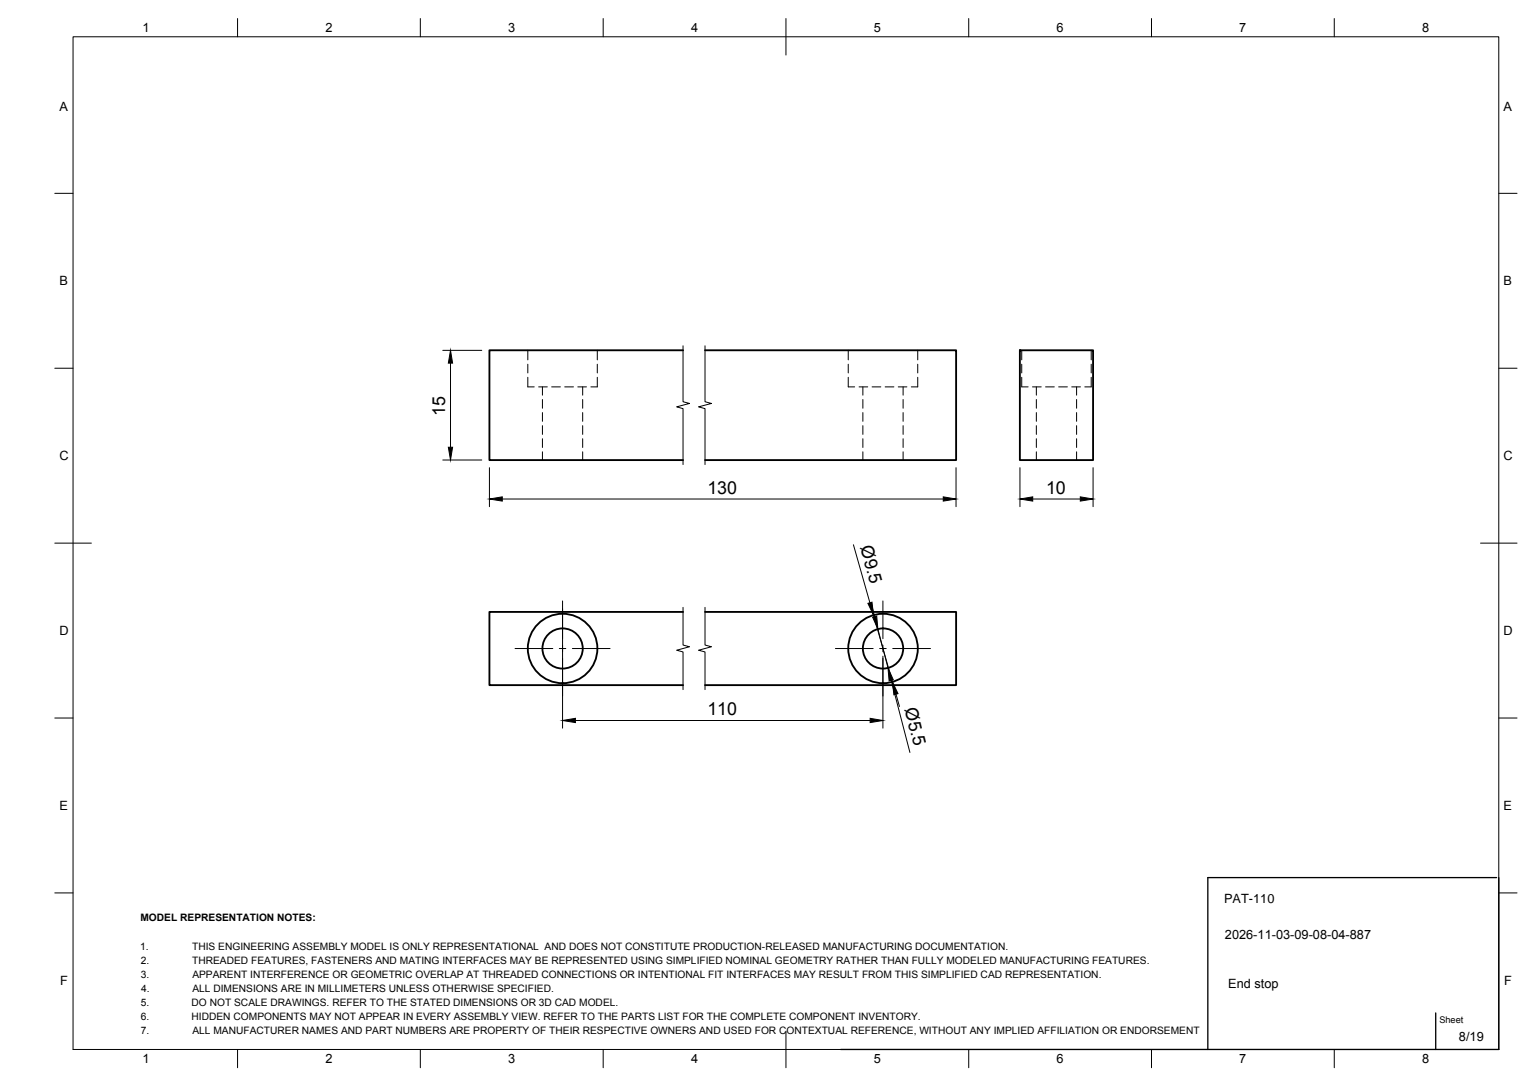
ISO-10303-21;
HEADER;
/* Generated by software containing ST-Developer
 * from STEP Tools, Inc. (www.steptools.com) 
 */

FILE_DESCRIPTION(
/* description */ ('Twin-shaft manual slide'),
/* implementation_level */ '2;1');

FILE_NAME(
/* name */ 'End stop.step',
/* time_stamp */ '2026-10-27T18:38:08-07:00',
/* author */ (''),
/* organization */ (''),
/* preprocessor_version */ 'ST-DEVELOPER v20.2',
/* originating_system */ 'Autodesk Translation Framework v15.17.0.0',
/* authorisation */ '');

FILE_SCHEMA (('AUTOMOTIVE_DESIGN { 1 0 10303 214 3 1 1 }'));
ENDSEC;

DATA;
#10=MECHANICAL_DESIGN_GEOMETRIC_PRESENTATION_REPRESENTATION('',(#280),#6463);
#248=SHAPE_REPRESENTATION_RELATIONSHIP('SRR','None',#6566,#264);
#264=ADVANCED_BREP_SHAPE_REPRESENTATION('',(#295),#6449);
#280=STYLED_ITEM('',(#6733),#295);
#295=MANIFOLD_SOLID_BREP('Body1',#3643);
#339=FACE_BOUND('',#832,.T.);
#340=FACE_BOUND('',#835,.T.);
#341=FACE_BOUND('',#843,.T.);
#342=FACE_BOUND('',#844,.T.);
#343=FACE_BOUND('',#846,.T.);
#344=FACE_BOUND('',#847,.T.);
#436=PLANE('',#3956);
#437=PLANE('',#3961);
#438=PLANE('',#3967);
#439=PLANE('',#3968);
#440=PLANE('',#3969);
#441=PLANE('',#3970);
#442=PLANE('',#3971);
#443=PLANE('',#3972);
#588=FACE_OUTER_BOUND('',#830,.T.);
#589=FACE_OUTER_BOUND('',#831,.T.);
#590=FACE_OUTER_BOUND('',#833,.T.);
#591=FACE_OUTER_BOUND('',#834,.T.);
#592=FACE_OUTER_BOUND('',#836,.T.);
#593=FACE_OUTER_BOUND('',#837,.T.);
#594=FACE_OUTER_BOUND('',#838,.T.);
#595=FACE_OUTER_BOUND('',#839,.T.);
#596=FACE_OUTER_BOUND('',#840,.T.);
#597=FACE_OUTER_BOUND('',#841,.T.);
#598=FACE_OUTER_BOUND('',#842,.T.);
#599=FACE_OUTER_BOUND('',#845,.T.);
#830=EDGE_LOOP('',(#2784,#2785,#2786,#2787));
#831=EDGE_LOOP('',(#2788));
#832=EDGE_LOOP('',(#2789));
#833=EDGE_LOOP('',(#2790,#2791,#2792,#2793));
#834=EDGE_LOOP('',(#2794));
#835=EDGE_LOOP('',(#2795));
#836=EDGE_LOOP('',(#2796,#2797,#2798,#2799));
#837=EDGE_LOOP('',(#2800,#2801,#2802,#2803));
#838=EDGE_LOOP('',(#2804,#2805,#2806,#2807));
#839=EDGE_LOOP('',(#2808,#2809,#2810,#2811));
#840=EDGE_LOOP('',(#2812,#2813,#2814,#2815));
#841=EDGE_LOOP('',(#2816,#2817,#2818,#2819));
#842=EDGE_LOOP('',(#2820,#2821,#2822,#2823));
#843=EDGE_LOOP('',(#2824));
#844=EDGE_LOOP('',(#2825));
#845=EDGE_LOOP('',(#2826,#2827,#2828,#2829));
#846=EDGE_LOOP('',(#2830));
#847=EDGE_LOOP('',(#2831));
#1136=LINE('',#5735,#1422);
#1137=LINE('',#5744,#1423);
#1138=LINE('',#5752,#1424);
#1139=LINE('',#5756,#1425);
#1140=LINE('',#5760,#1426);
#1141=LINE('',#5762,#1427);
#1142=LINE('',#5764,#1428);
#1143=LINE('',#5765,#1429);
#1144=LINE('',#5768,#1430);
#1145=LINE('',#5770,#1431);
#1146=LINE('',#5771,#1432);
#1147=LINE('',#5774,#1433);
#1148=LINE('',#5776,#1434);
#1149=LINE('',#5777,#1435);
#1150=LINE('',#5779,#1436);
#1151=LINE('',#5780,#1437);
#1422=VECTOR('',#4606,0.475);
#1423=VECTOR('',#4617,0.475);
#1424=VECTOR('',#4628,0.275);
#1425=VECTOR('',#4633,0.275);
#1426=VECTOR('',#4636,1.);
#1427=VECTOR('',#4637,1.);
#1428=VECTOR('',#4638,1.);
#1429=VECTOR('',#4639,1.);
#1430=VECTOR('',#4642,1.);
#1431=VECTOR('',#4643,1.);
#1432=VECTOR('',#4644,1.);
#1433=VECTOR('',#4647,1.);
#1434=VECTOR('',#4648,1.);
#1435=VECTOR('',#4649,1.);
#1436=VECTOR('',#4652,1.);
#1437=VECTOR('',#4653,1.);
#1658=CIRCLE('',#3954,0.475);
#1659=CIRCLE('',#3955,0.475);
#1660=CIRCLE('',#3957,0.275);
#1661=CIRCLE('',#3959,0.475);
#1662=CIRCLE('',#3960,0.475);
#1663=CIRCLE('',#3962,0.275);
#1664=CIRCLE('',#3964,0.275);
#1665=CIRCLE('',#3966,0.275);
#1859=VERTEX_POINT('',#5732);
#1860=VERTEX_POINT('',#5734);
#1861=VERTEX_POINT('',#5738);
#1862=VERTEX_POINT('',#5741);
#1863=VERTEX_POINT('',#5743);
#1864=VERTEX_POINT('',#5747);
#1865=VERTEX_POINT('',#5750);
#1866=VERTEX_POINT('',#5754);
#1867=VERTEX_POINT('',#5758);
#1868=VERTEX_POINT('',#5759);
#1869=VERTEX_POINT('',#5761);
#1870=VERTEX_POINT('',#5763);
#1871=VERTEX_POINT('',#5767);
#1872=VERTEX_POINT('',#5769);
#1873=VERTEX_POINT('',#5773);
#1874=VERTEX_POINT('',#5775);
#2197=EDGE_CURVE('',#1859,#1859,#1658,.T.);
#2198=EDGE_CURVE('',#1859,#1860,#1136,.T.);
#2199=EDGE_CURVE('',#1860,#1860,#1659,.T.);
#2200=EDGE_CURVE('',#1861,#1861,#1660,.T.);
#2201=EDGE_CURVE('',#1862,#1862,#1661,.T.);
#2202=EDGE_CURVE('',#1862,#1863,#1137,.T.);
#2203=EDGE_CURVE('',#1863,#1863,#1662,.T.);
#2204=EDGE_CURVE('',#1864,#1864,#1663,.T.);
#2205=EDGE_CURVE('',#1865,#1865,#1664,.T.);
#2206=EDGE_CURVE('',#1865,#1861,#1138,.T.);
#2207=EDGE_CURVE('',#1866,#1866,#1665,.T.);
#2208=EDGE_CURVE('',#1866,#1864,#1139,.T.);
#2209=EDGE_CURVE('',#1867,#1868,#1140,.T.);
#2210=EDGE_CURVE('',#1868,#1869,#1141,.T.);
#2211=EDGE_CURVE('',#1870,#1869,#1142,.T.);
#2212=EDGE_CURVE('',#1867,#1870,#1143,.T.);
#2213=EDGE_CURVE('',#1871,#1867,#1144,.T.);
#2214=EDGE_CURVE('',#1872,#1870,#1145,.T.);
#2215=EDGE_CURVE('',#1871,#1872,#1146,.T.);
#2216=EDGE_CURVE('',#1873,#1871,#1147,.T.);
#2217=EDGE_CURVE('',#1874,#1872,#1148,.T.);
#2218=EDGE_CURVE('',#1873,#1874,#1149,.T.);
#2219=EDGE_CURVE('',#1868,#1873,#1150,.T.);
#2220=EDGE_CURVE('',#1869,#1874,#1151,.T.);
#2784=ORIENTED_EDGE('',*,*,#2197,.F.);
#2785=ORIENTED_EDGE('',*,*,#2198,.T.);
#2786=ORIENTED_EDGE('',*,*,#2199,.F.);
#2787=ORIENTED_EDGE('',*,*,#2198,.F.);
#2788=ORIENTED_EDGE('',*,*,#2197,.T.);
#2789=ORIENTED_EDGE('',*,*,#2200,.F.);
#2790=ORIENTED_EDGE('',*,*,#2201,.F.);
#2791=ORIENTED_EDGE('',*,*,#2202,.T.);
#2792=ORIENTED_EDGE('',*,*,#2203,.F.);
#2793=ORIENTED_EDGE('',*,*,#2202,.F.);
#2794=ORIENTED_EDGE('',*,*,#2201,.T.);
#2795=ORIENTED_EDGE('',*,*,#2204,.F.);
#2796=ORIENTED_EDGE('',*,*,#2205,.F.);
#2797=ORIENTED_EDGE('',*,*,#2206,.T.);
#2798=ORIENTED_EDGE('',*,*,#2200,.T.);
#2799=ORIENTED_EDGE('',*,*,#2206,.F.);
#2800=ORIENTED_EDGE('',*,*,#2207,.F.);
#2801=ORIENTED_EDGE('',*,*,#2208,.T.);
#2802=ORIENTED_EDGE('',*,*,#2204,.T.);
#2803=ORIENTED_EDGE('',*,*,#2208,.F.);
#2804=ORIENTED_EDGE('',*,*,#2209,.T.);
#2805=ORIENTED_EDGE('',*,*,#2210,.T.);
#2806=ORIENTED_EDGE('',*,*,#2211,.F.);
#2807=ORIENTED_EDGE('',*,*,#2212,.F.);
#2808=ORIENTED_EDGE('',*,*,#2213,.T.);
#2809=ORIENTED_EDGE('',*,*,#2212,.T.);
#2810=ORIENTED_EDGE('',*,*,#2214,.F.);
#2811=ORIENTED_EDGE('',*,*,#2215,.F.);
#2812=ORIENTED_EDGE('',*,*,#2216,.T.);
#2813=ORIENTED_EDGE('',*,*,#2215,.T.);
#2814=ORIENTED_EDGE('',*,*,#2217,.F.);
#2815=ORIENTED_EDGE('',*,*,#2218,.F.);
#2816=ORIENTED_EDGE('',*,*,#2219,.T.);
#2817=ORIENTED_EDGE('',*,*,#2218,.T.);
#2818=ORIENTED_EDGE('',*,*,#2220,.F.);
#2819=ORIENTED_EDGE('',*,*,#2210,.F.);
#2820=ORIENTED_EDGE('',*,*,#2220,.T.);
#2821=ORIENTED_EDGE('',*,*,#2217,.T.);
#2822=ORIENTED_EDGE('',*,*,#2214,.T.);
#2823=ORIENTED_EDGE('',*,*,#2211,.T.);
#2824=ORIENTED_EDGE('',*,*,#2199,.T.);
#2825=ORIENTED_EDGE('',*,*,#2203,.T.);
#2826=ORIENTED_EDGE('',*,*,#2219,.F.);
#2827=ORIENTED_EDGE('',*,*,#2209,.F.);
#2828=ORIENTED_EDGE('',*,*,#2213,.F.);
#2829=ORIENTED_EDGE('',*,*,#2216,.F.);
#2830=ORIENTED_EDGE('',*,*,#2205,.T.);
#2831=ORIENTED_EDGE('',*,*,#2207,.T.);
#3388=CYLINDRICAL_SURFACE('',#3953,0.475);
#3389=CYLINDRICAL_SURFACE('',#3958,0.475);
#3390=CYLINDRICAL_SURFACE('',#3963,0.275);
#3391=CYLINDRICAL_SURFACE('',#3965,0.275);
#3493=ADVANCED_FACE('',(#588),#3388,.F.);
#3494=ADVANCED_FACE('',(#589,#339),#436,.T.);
#3495=ADVANCED_FACE('',(#590),#3389,.F.);
#3496=ADVANCED_FACE('',(#591,#340),#437,.T.);
#3497=ADVANCED_FACE('',(#592),#3390,.F.);
#3498=ADVANCED_FACE('',(#593),#3391,.F.);
#3499=ADVANCED_FACE('',(#594),#438,.T.);
#3500=ADVANCED_FACE('',(#595),#439,.T.);
#3501=ADVANCED_FACE('',(#596),#440,.T.);
#3502=ADVANCED_FACE('',(#597),#441,.T.);
#3503=ADVANCED_FACE('',(#598,#341,#342),#442,.T.);
#3504=ADVANCED_FACE('',(#599,#343,#344),#443,.F.);
#3643=CLOSED_SHELL('',(#3493,#3494,#3495,#3496,#3497,#3498,#3499,#3500,
#3501,#3502,#3503,#3504));
#3952=AXIS2_PLACEMENT_3D('',#5730,#4600,#4601);
#3953=AXIS2_PLACEMENT_3D('',#5731,#4602,#4603);
#3954=AXIS2_PLACEMENT_3D('',#5733,#4604,#4605);
#3955=AXIS2_PLACEMENT_3D('',#5736,#4607,#4608);
#3956=AXIS2_PLACEMENT_3D('',#5737,#4609,#4610);
#3957=AXIS2_PLACEMENT_3D('',#5739,#4611,#4612);
#3958=AXIS2_PLACEMENT_3D('',#5740,#4613,#4614);
#3959=AXIS2_PLACEMENT_3D('',#5742,#4615,#4616);
#3960=AXIS2_PLACEMENT_3D('',#5745,#4618,#4619);
#3961=AXIS2_PLACEMENT_3D('',#5746,#4620,#4621);
#3962=AXIS2_PLACEMENT_3D('',#5748,#4622,#4623);
#3963=AXIS2_PLACEMENT_3D('',#5749,#4624,#4625);
#3964=AXIS2_PLACEMENT_3D('',#5751,#4626,#4627);
#3965=AXIS2_PLACEMENT_3D('',#5753,#4629,#4630);
#3966=AXIS2_PLACEMENT_3D('',#5755,#4631,#4632);
#3967=AXIS2_PLACEMENT_3D('',#5757,#4634,#4635);
#3968=AXIS2_PLACEMENT_3D('',#5766,#4640,#4641);
#3969=AXIS2_PLACEMENT_3D('',#5772,#4645,#4646);
#3970=AXIS2_PLACEMENT_3D('',#5778,#4650,#4651);
#3971=AXIS2_PLACEMENT_3D('',#5781,#4654,#4655);
#3972=AXIS2_PLACEMENT_3D('',#5782,#4656,#4657);
#4600=DIRECTION('axis',(0.,0.,1.));
#4601=DIRECTION('refdir',(1.,0.,0.));
#4602=DIRECTION('center_axis',(0.,0.,1.));
#4603=DIRECTION('ref_axis',(1.,0.,0.));
#4604=DIRECTION('center_axis',(0.,0.,1.));
#4605=DIRECTION('ref_axis',(1.,0.,0.));
#4606=DIRECTION('',(0.,0.,1.));
#4607=DIRECTION('center_axis',(0.,0.,-1.));
#4608=DIRECTION('ref_axis',(1.,0.,0.));
#4609=DIRECTION('center_axis',(0.,0.,1.));
#4610=DIRECTION('ref_axis',(1.,0.,0.));
#4611=DIRECTION('center_axis',(0.,0.,1.));
#4612=DIRECTION('ref_axis',(1.,0.,0.));
#4613=DIRECTION('center_axis',(0.,0.,1.));
#4614=DIRECTION('ref_axis',(1.,0.,0.));
#4615=DIRECTION('center_axis',(0.,0.,1.));
#4616=DIRECTION('ref_axis',(1.,0.,0.));
#4617=DIRECTION('',(0.,0.,1.));
#4618=DIRECTION('center_axis',(0.,0.,-1.));
#4619=DIRECTION('ref_axis',(1.,0.,0.));
#4620=DIRECTION('center_axis',(0.,0.,1.));
#4621=DIRECTION('ref_axis',(1.,0.,0.));
#4622=DIRECTION('center_axis',(0.,0.,1.));
#4623=DIRECTION('ref_axis',(1.,0.,0.));
#4624=DIRECTION('center_axis',(0.,0.,1.));
#4625=DIRECTION('ref_axis',(1.,0.,0.));
#4626=DIRECTION('center_axis',(0.,0.,1.));
#4627=DIRECTION('ref_axis',(1.,0.,0.));
#4628=DIRECTION('',(0.,0.,1.));
#4629=DIRECTION('center_axis',(0.,0.,1.));
#4630=DIRECTION('ref_axis',(1.,0.,0.));
#4631=DIRECTION('center_axis',(0.,0.,1.));
#4632=DIRECTION('ref_axis',(1.,0.,0.));
#4633=DIRECTION('',(0.,0.,1.));
#4634=DIRECTION('center_axis',(0.,1.,0.));
#4635=DIRECTION('ref_axis',(-1.,0.,0.));
#4636=DIRECTION('',(-1.,0.,0.));
#4637=DIRECTION('',(0.,0.,1.));
#4638=DIRECTION('',(-1.,0.,0.));
#4639=DIRECTION('',(0.,0.,1.));
#4640=DIRECTION('center_axis',(1.,0.,0.));
#4641=DIRECTION('ref_axis',(0.,1.,0.));
#4642=DIRECTION('',(0.,1.,0.));
#4643=DIRECTION('',(0.,1.,0.));
#4644=DIRECTION('',(0.,0.,1.));
#4645=DIRECTION('center_axis',(0.,-1.,0.));
#4646=DIRECTION('ref_axis',(1.,0.,0.));
#4647=DIRECTION('',(1.,0.,0.));
#4648=DIRECTION('',(1.,0.,0.));
#4649=DIRECTION('',(0.,0.,1.));
#4650=DIRECTION('center_axis',(-1.,0.,0.));
#4651=DIRECTION('ref_axis',(0.,-1.,0.));
#4652=DIRECTION('',(0.,-1.,0.));
#4653=DIRECTION('',(0.,-1.,0.));
#4654=DIRECTION('center_axis',(0.,0.,1.));
#4655=DIRECTION('ref_axis',(1.,0.,0.));
#4656=DIRECTION('center_axis',(0.,0.,1.));
#4657=DIRECTION('ref_axis',(1.,0.,0.));
#5730=CARTESIAN_POINT('',(0.,0.,0.));
#5731=CARTESIAN_POINT('Origin',(3.5,-5.5,2.));
#5732=CARTESIAN_POINT('',(3.025,-5.5,2.));
#5733=CARTESIAN_POINT('Origin',(3.5,-5.5,2.));
#5734=CARTESIAN_POINT('',(3.025,-5.5,2.5));
#5735=CARTESIAN_POINT('',(3.025,-5.5,2.));
#5736=CARTESIAN_POINT('Origin',(3.5,-5.5,2.5));
#5737=CARTESIAN_POINT('Origin',(3.5,-5.5,2.));
#5738=CARTESIAN_POINT('',(3.225,-5.5,2.));
#5739=CARTESIAN_POINT('Origin',(3.5,-5.5,2.));
#5740=CARTESIAN_POINT('Origin',(3.5,5.5,2.));
#5741=CARTESIAN_POINT('',(3.025,5.5,2.));
#5742=CARTESIAN_POINT('Origin',(3.5,5.5,2.));
#5743=CARTESIAN_POINT('',(3.025,5.5,2.5));
#5744=CARTESIAN_POINT('',(3.025,5.5,2.));
#5745=CARTESIAN_POINT('Origin',(3.5,5.5,2.5));
#5746=CARTESIAN_POINT('Origin',(3.5,5.5,2.));
#5747=CARTESIAN_POINT('',(3.225,5.5,2.));
#5748=CARTESIAN_POINT('Origin',(3.5,5.5,2.));
#5749=CARTESIAN_POINT('Origin',(3.5,-5.5,0.9));
#5750=CARTESIAN_POINT('',(3.225,-5.5,1.));
#5751=CARTESIAN_POINT('Origin',(3.5,-5.5,1.));
#5752=CARTESIAN_POINT('',(3.225,-5.5,0.9));
#5753=CARTESIAN_POINT('Origin',(3.5,5.5,0.9));
#5754=CARTESIAN_POINT('',(3.225,5.5,1.));
#5755=CARTESIAN_POINT('Origin',(3.5,5.5,1.));
#5756=CARTESIAN_POINT('',(3.225,5.5,0.9));
#5757=CARTESIAN_POINT('Origin',(4.,6.5,1.));
#5758=CARTESIAN_POINT('',(4.,6.5,1.));
#5759=CARTESIAN_POINT('',(3.,6.5,1.));
#5760=CARTESIAN_POINT('',(4.,6.5,1.));
#5761=CARTESIAN_POINT('',(3.,6.5,2.5));
#5762=CARTESIAN_POINT('',(3.,6.5,1.));
#5763=CARTESIAN_POINT('',(4.,6.5,2.5));
#5764=CARTESIAN_POINT('',(4.,6.5,2.5));
#5765=CARTESIAN_POINT('',(4.,6.5,1.));
#5766=CARTESIAN_POINT('Origin',(4.,-6.5,1.));
#5767=CARTESIAN_POINT('',(4.,-6.5,1.));
#5768=CARTESIAN_POINT('',(4.,-6.5,1.));
#5769=CARTESIAN_POINT('',(4.,-6.5,2.5));
#5770=CARTESIAN_POINT('',(4.,-6.5,2.5));
#5771=CARTESIAN_POINT('',(4.,-6.5,1.));
#5772=CARTESIAN_POINT('Origin',(3.,-6.5,1.));
#5773=CARTESIAN_POINT('',(3.,-6.5,1.));
#5774=CARTESIAN_POINT('',(3.,-6.5,1.));
#5775=CARTESIAN_POINT('',(3.,-6.5,2.5));
#5776=CARTESIAN_POINT('',(3.,-6.5,2.5));
#5777=CARTESIAN_POINT('',(3.,-6.5,1.));
#5778=CARTESIAN_POINT('Origin',(3.,6.5,1.));
#5779=CARTESIAN_POINT('',(3.,6.5,1.));
#5780=CARTESIAN_POINT('',(3.,6.5,2.5));
#5781=CARTESIAN_POINT('Origin',(3.5,0.,2.5));
#5782=CARTESIAN_POINT('Origin',(3.5,0.,1.));
#6428=UNCERTAINTY_MEASURE_WITH_UNIT(LENGTH_MEASURE(0.001),#6464,
'DISTANCE_ACCURACY_VALUE',
'Maximum model space distance between geometric entities at asserted c
onnectivities');
#6442=UNCERTAINTY_MEASURE_WITH_UNIT(LENGTH_MEASURE(0.001),#6464,
'DISTANCE_ACCURACY_VALUE',
'Maximum model space distance between geometric entities at asserted c
onnectivities');
#6449=(
GEOMETRIC_REPRESENTATION_CONTEXT(3)
GLOBAL_UNCERTAINTY_ASSIGNED_CONTEXT((#6428))
GLOBAL_UNIT_ASSIGNED_CONTEXT((#6464,#6466,#6467))
REPRESENTATION_CONTEXT('','3D')
);
#6463=(
GEOMETRIC_REPRESENTATION_CONTEXT(3)
GLOBAL_UNCERTAINTY_ASSIGNED_CONTEXT((#6442))
GLOBAL_UNIT_ASSIGNED_CONTEXT((#6464,#6466,#6467))
REPRESENTATION_CONTEXT('','3D')
);
#6464=(
LENGTH_UNIT()
NAMED_UNIT(*)
SI_UNIT(.CENTI.,.METRE.)
);
#6466=(
NAMED_UNIT(*)
PLANE_ANGLE_UNIT()
SI_UNIT($,.RADIAN.)
);
#6467=(
NAMED_UNIT(*)
SI_UNIT($,.STERADIAN.)
SOLID_ANGLE_UNIT()
);
#6474=SHAPE_DEFINITION_REPRESENTATION(#6494,#6566);
#6494=PRODUCT_DEFINITION_SHAPE('',$,#6587);
#6566=SHAPE_REPRESENTATION('',(#3952),#6449);
#6580=PRODUCT_DEFINITION_CONTEXT('part definition',#6642,'design');
#6587=PRODUCT_DEFINITION('End stop','End stop',#6607,#6580);
#6607=PRODUCT_DEFINITION_FORMATION('',$,#6650);
#6642=APPLICATION_CONTEXT(
'Core Data for Automotive Mechanical Design Process');
#6643=PRODUCT_CONTEXT('part definition',#6642,'mechanical');
#6650=PRODUCT('End stop','End stop','End stop',(#6643));
#6727=COLOUR_RGB('Sky Blue',0.24,0.69,0.87);
#6728=FILL_AREA_STYLE_COLOUR('',#6727);
#6729=FILL_AREA_STYLE('',(#6728));
#6730=SURFACE_STYLE_FILL_AREA(#6729);
#6731=SURFACE_SIDE_STYLE('',(#6730));
#6732=SURFACE_STYLE_USAGE(.BOTH.,#6731);
#6733=PRESENTATION_STYLE_ASSIGNMENT((#6732));
ENDSEC;
END-ISO-10303-21;
